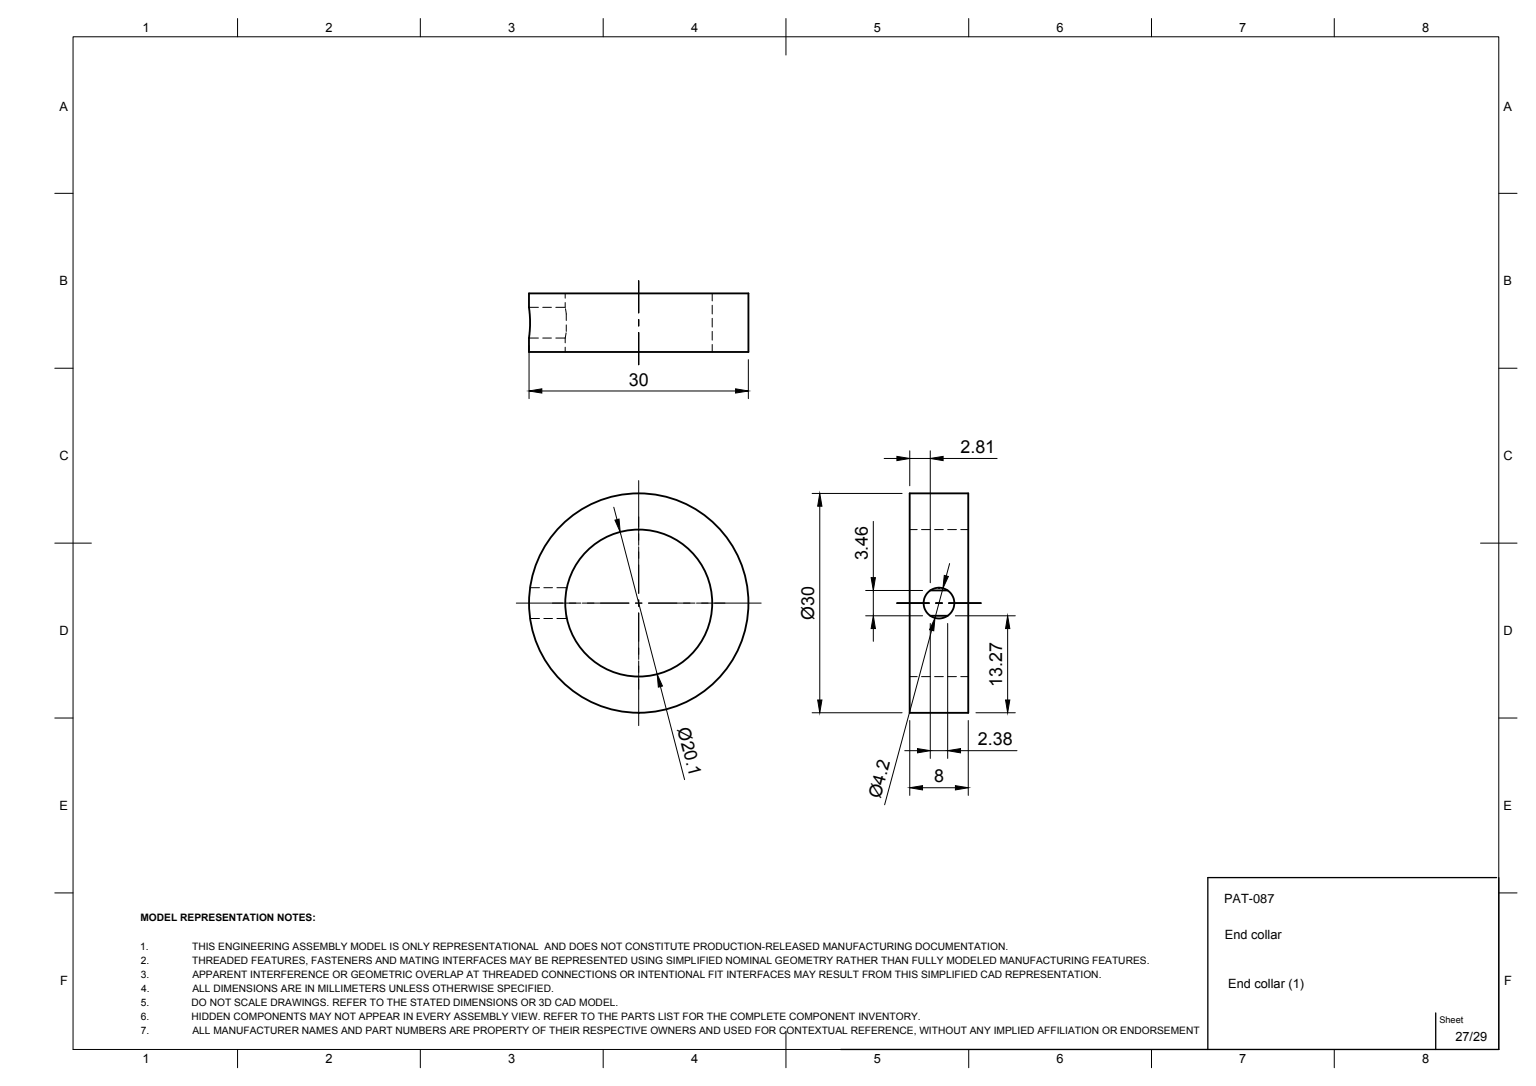
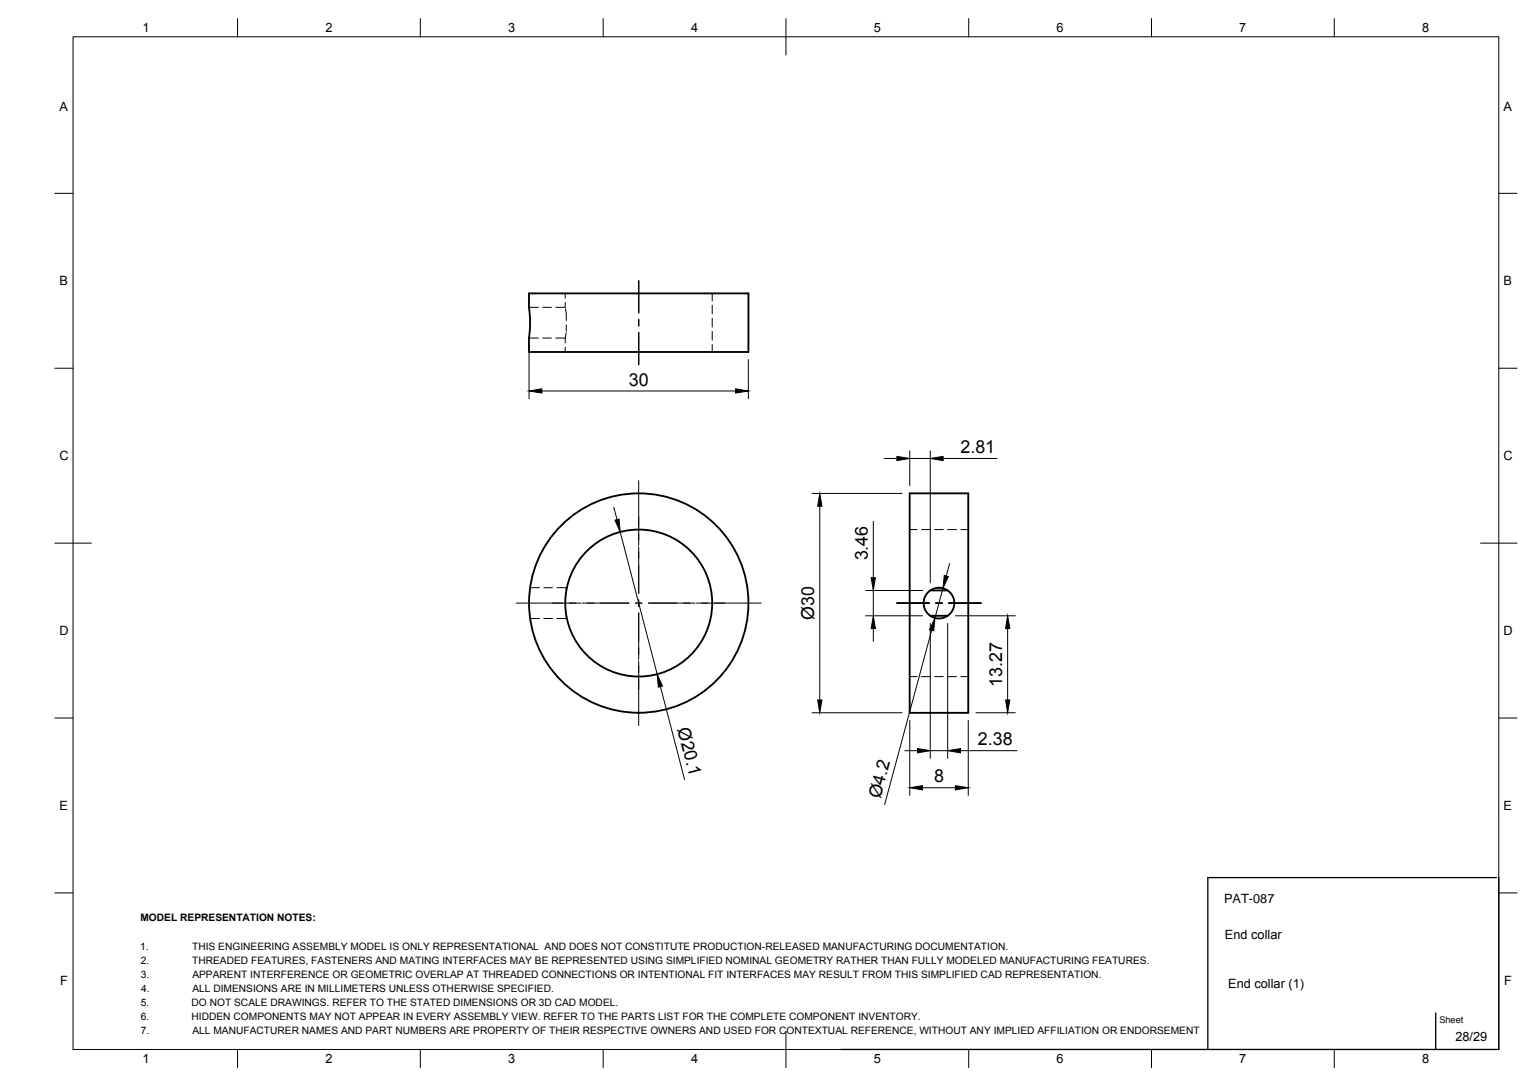
ISO-10303-21;
HEADER;
/* Generated by software containing ST-Developer
 * from STEP Tools, Inc. (www.steptools.com) 
 */

FILE_DESCRIPTION(
/* description */ ('Rigid flange shaft coupling assembly'),
/* implementation_level */ '2;1');

FILE_NAME(
/* name */ 'End collar.step',
/* time_stamp */ '2026-10-27T10:47:16-07:00',
/* author */ (''),
/* organization */ (''),
/* preprocessor_version */ 'ST-DEVELOPER v20.2',
/* originating_system */ 'Autodesk Translation Framework v15.17.0.0',
/* authorisation */ '');

FILE_SCHEMA (('AUTOMOTIVE_DESIGN { 1 0 10303 214 3 1 1 }'));
ENDSEC;

DATA;
#10=MECHANICAL_DESIGN_GEOMETRIC_PRESENTATION_REPRESENTATION('',(#419),#9141);
#332=B_SPLINE_CURVE_WITH_KNOTS('',3,(#8495,#8496,#8497,#8498,#8499,#8500,
#8501,#8502,#8503,#8504,#8505,#8506,#8507,#8508),.UNSPECIFIED.,.F.,.F.,
(4,2,2,2,2,2,4),(0.75600573798702,0.793568827564647,0.872922520054201,0.952276212543756,
1.03162990503331,1.11098359752287,1.14854668710049),.UNSPECIFIED.);
#333=B_SPLINE_CURVE_WITH_KNOTS('',3,(#8514,#8515,#8516,#8517,#8518,#8519,
#8520,#8521,#8522,#8523,#8524,#8525,#8526,#8527,#8528,#8529,#8530,#8531),
 .UNSPECIFIED.,.F.,.F.,(4,2,2,2,2,2,2,2,4),(0.,0.079216580773363,0.158433161546726,
0.23764869707457,0.316864232602414,0.396079768130259,0.475295303658103,
0.554511884431466,0.633728465204829),.UNSPECIFIED.);
#334=B_SPLINE_CURVE_WITH_KNOTS('',3,(#8532,#8533,#8534,#8535,#8536,#8537,
#8538,#8539,#8540,#8541,#8542,#8543,#8544,#8545,#8546,#8547,#8548,#8549),
 .UNSPECIFIED.,.F.,.F.,(4,2,2,2,2,2,2,2,4),(0.633728465204829,0.712945045978192,
0.792161626751555,0.871377162279399,0.950592697807243,1.02980823333509,
1.10902376886293,1.18824034963629,1.26745693040966),.UNSPECIFIED.);
#335=B_SPLINE_CURVE_WITH_KNOTS('',3,(#8552,#8553,#8554,#8555,#8556,#8557,
#8558,#8559,#8560,#8561,#8562,#8563,#8564,#8565),.UNSPECIFIED.,.F.,.F.,
(4,2,2,2,2,2,4),(0.121154929624515,0.158718019202143,0.238071711691697,
0.317425404181252,0.396779096670807,0.476132789160362,0.513695878737989),
 .UNSPECIFIED.);
#362=SHAPE_REPRESENTATION_RELATIONSHIP('SRR','None',#9298,#390);
#390=ADVANCED_BREP_SHAPE_REPRESENTATION('',(#447),#9133);
#419=STYLED_ITEM('',(#9486),#447);
#447=MANIFOLD_SOLID_BREP('Body1',#4774);
#555=FACE_BOUND('',#1309,.T.);
#556=FACE_BOUND('',#1311,.T.);
#557=FACE_BOUND('',#1313,.T.);
#558=FACE_BOUND('',#1315,.T.);
#685=PLANE('',#5446);
#686=PLANE('',#5451);
#687=PLANE('',#5458);
#688=PLANE('',#5459);
#931=FACE_OUTER_BOUND('',#1305,.T.);
#932=FACE_OUTER_BOUND('',#1306,.T.);
#933=FACE_OUTER_BOUND('',#1307,.T.);
#934=FACE_OUTER_BOUND('',#1308,.T.);
#935=FACE_OUTER_BOUND('',#1310,.T.);
#936=FACE_OUTER_BOUND('',#1312,.T.);
#937=FACE_OUTER_BOUND('',#1314,.T.);
#1305=EDGE_LOOP('',(#4047,#4048));
#1306=EDGE_LOOP('',(#4049,#4050,#4051,#4052,#4053,#4054,#4055,#4056,#4057));
#1307=EDGE_LOOP('',(#4058,#4059,#4060));
#1308=EDGE_LOOP('',(#4061,#4062,#4063,#4064));
#1309=EDGE_LOOP('',(#4065,#4066,#4067,#4068));
#1310=EDGE_LOOP('',(#4069,#4070,#4071,#4072));
#1311=EDGE_LOOP('',(#4073,#4074));
#1312=EDGE_LOOP('',(#4075));
#1313=EDGE_LOOP('',(#4076));
#1314=EDGE_LOOP('',(#4077));
#1315=EDGE_LOOP('',(#4078));
#1636=LINE('',#8491,#1981);
#1637=LINE('',#8512,#1982);
#1638=LINE('',#8567,#1983);
#1639=LINE('',#8572,#1984);
#1640=LINE('',#8578,#1985);
#1981=VECTOR('',#6581,1.);
#1982=VECTOR('',#6588,0.21);
#1983=VECTOR('',#6593,1.);
#1984=VECTOR('',#6598,1.005);
#1985=VECTOR('',#6605,1.5);
#2234=CIRCLE('',#5447,0.21);
#2235=CIRCLE('',#5449,0.21);
#2236=CIRCLE('',#5450,0.21);
#2237=CIRCLE('',#5453,1.005);
#2238=CIRCLE('',#5454,1.005);
#2239=CIRCLE('',#5456,1.5);
#2240=CIRCLE('',#5457,1.5);
#2551=VERTEX_POINT('',#8489);
#2552=VERTEX_POINT('',#8490);
#2553=VERTEX_POINT('',#8494);
#2554=VERTEX_POINT('',#8509);
#2555=VERTEX_POINT('',#8511);
#2556=VERTEX_POINT('',#8513);
#2557=VERTEX_POINT('',#8550);
#2558=VERTEX_POINT('',#8569);
#2559=VERTEX_POINT('',#8571);
#2560=VERTEX_POINT('',#8575);
#2561=VERTEX_POINT('',#8577);
#3067=EDGE_CURVE('',#2551,#2552,#1636,.T.);
#3068=EDGE_CURVE('',#2551,#2552,#2234,.T.);
#3069=EDGE_CURVE('',#2553,#2551,#332,.T.);
#3070=EDGE_CURVE('',#2554,#2553,#2235,.T.);
#3071=EDGE_CURVE('',#2554,#2555,#1637,.T.);
#3072=EDGE_CURVE('',#2556,#2555,#333,.T.);
#3073=EDGE_CURVE('',#2555,#2556,#334,.T.);
#3074=EDGE_CURVE('',#2557,#2554,#2236,.T.);
#3075=EDGE_CURVE('',#2552,#2557,#335,.T.);
#3076=EDGE_CURVE('',#2557,#2553,#1638,.T.);
#3077=EDGE_CURVE('',#2558,#2558,#2237,.T.);
#3078=EDGE_CURVE('',#2558,#2559,#1639,.T.);
#3079=EDGE_CURVE('',#2559,#2559,#2238,.T.);
#3080=EDGE_CURVE('',#2560,#2560,#2239,.T.);
#3081=EDGE_CURVE('',#2560,#2561,#1640,.T.);
#3082=EDGE_CURVE('',#2561,#2561,#2240,.T.);
#4047=ORIENTED_EDGE('',*,*,#3067,.F.);
#4048=ORIENTED_EDGE('',*,*,#3068,.T.);
#4049=ORIENTED_EDGE('',*,*,#3069,.F.);
#4050=ORIENTED_EDGE('',*,*,#3070,.F.);
#4051=ORIENTED_EDGE('',*,*,#3071,.T.);
#4052=ORIENTED_EDGE('',*,*,#3072,.F.);
#4053=ORIENTED_EDGE('',*,*,#3073,.F.);
#4054=ORIENTED_EDGE('',*,*,#3071,.F.);
#4055=ORIENTED_EDGE('',*,*,#3074,.F.);
#4056=ORIENTED_EDGE('',*,*,#3075,.F.);
#4057=ORIENTED_EDGE('',*,*,#3068,.F.);
#4058=ORIENTED_EDGE('',*,*,#3076,.F.);
#4059=ORIENTED_EDGE('',*,*,#3074,.T.);
#4060=ORIENTED_EDGE('',*,*,#3070,.T.);
#4061=ORIENTED_EDGE('',*,*,#3077,.F.);
#4062=ORIENTED_EDGE('',*,*,#3078,.T.);
#4063=ORIENTED_EDGE('',*,*,#3079,.T.);
#4064=ORIENTED_EDGE('',*,*,#3078,.F.);
#4065=ORIENTED_EDGE('',*,*,#3075,.T.);
#4066=ORIENTED_EDGE('',*,*,#3076,.T.);
#4067=ORIENTED_EDGE('',*,*,#3069,.T.);
#4068=ORIENTED_EDGE('',*,*,#3067,.T.);
#4069=ORIENTED_EDGE('',*,*,#3080,.F.);
#4070=ORIENTED_EDGE('',*,*,#3081,.T.);
#4071=ORIENTED_EDGE('',*,*,#3082,.T.);
#4072=ORIENTED_EDGE('',*,*,#3081,.F.);
#4073=ORIENTED_EDGE('',*,*,#3072,.T.);
#4074=ORIENTED_EDGE('',*,*,#3073,.T.);
#4075=ORIENTED_EDGE('',*,*,#3080,.T.);
#4076=ORIENTED_EDGE('',*,*,#3077,.T.);
#4077=ORIENTED_EDGE('',*,*,#3082,.F.);
#4078=ORIENTED_EDGE('',*,*,#3079,.F.);
#4466=CYLINDRICAL_SURFACE('',#5448,0.21);
#4467=CYLINDRICAL_SURFACE('',#5452,1.005);
#4468=CYLINDRICAL_SURFACE('',#5455,1.5);
#4667=ADVANCED_FACE('',(#931),#685,.T.);
#4668=ADVANCED_FACE('',(#932),#4466,.F.);
#4669=ADVANCED_FACE('',(#933),#686,.T.);
#4670=ADVANCED_FACE('',(#934,#555),#4467,.F.);
#4671=ADVANCED_FACE('',(#935,#556),#4468,.T.);
#4672=ADVANCED_FACE('',(#936,#557),#687,.T.);
#4673=ADVANCED_FACE('',(#937,#558),#688,.F.);
#4774=CLOSED_SHELL('',(#4667,#4668,#4669,#4670,#4671,#4672,#4673));
#5445=AXIS2_PLACEMENT_3D('',#8487,#6577,#6578);
#5446=AXIS2_PLACEMENT_3D('',#8488,#6579,#6580);
#5447=AXIS2_PLACEMENT_3D('',#8492,#6582,#6583);
#5448=AXIS2_PLACEMENT_3D('',#8493,#6584,#6585);
#5449=AXIS2_PLACEMENT_3D('',#8510,#6586,#6587);
#5450=AXIS2_PLACEMENT_3D('',#8551,#6589,#6590);
#5451=AXIS2_PLACEMENT_3D('',#8566,#6591,#6592);
#5452=AXIS2_PLACEMENT_3D('',#8568,#6594,#6595);
#5453=AXIS2_PLACEMENT_3D('',#8570,#6596,#6597);
#5454=AXIS2_PLACEMENT_3D('',#8573,#6599,#6600);
#5455=AXIS2_PLACEMENT_3D('',#8574,#6601,#6602);
#5456=AXIS2_PLACEMENT_3D('',#8576,#6603,#6604);
#5457=AXIS2_PLACEMENT_3D('',#8579,#6606,#6607);
#5458=AXIS2_PLACEMENT_3D('',#8580,#6608,#6609);
#5459=AXIS2_PLACEMENT_3D('',#8581,#6610,#6611);
#6577=DIRECTION('axis',(0.,0.,1.));
#6578=DIRECTION('refdir',(1.,0.,0.));
#6579=DIRECTION('center_axis',(0.,0.,1.));
#6580=DIRECTION('ref_axis',(1.,0.,0.));
#6581=DIRECTION('',(0.,1.,0.));
#6582=DIRECTION('center_axis',(0.,0.,1.));
#6583=DIRECTION('ref_axis',(1.,0.,0.));
#6584=DIRECTION('center_axis',(0.,0.,1.));
#6585=DIRECTION('ref_axis',(1.,0.,0.));
#6586=DIRECTION('center_axis',(0.,0.,1.));
#6587=DIRECTION('ref_axis',(1.,0.,0.));
#6588=DIRECTION('',(0.,0.,1.));
#6589=DIRECTION('center_axis',(0.,0.,1.));
#6590=DIRECTION('ref_axis',(1.,0.,0.));
#6591=DIRECTION('center_axis',(0.,0.,1.));
#6592=DIRECTION('ref_axis',(1.,0.,0.));
#6593=DIRECTION('',(0.,-1.,0.));
#6594=DIRECTION('center_axis',(0.,1.,0.));
#6595=DIRECTION('ref_axis',(1.,0.,0.));
#6596=DIRECTION('center_axis',(0.,-1.,0.));
#6597=DIRECTION('ref_axis',(1.,0.,0.));
#6598=DIRECTION('',(0.,-1.,0.));
#6599=DIRECTION('center_axis',(0.,-1.,0.));
#6600=DIRECTION('ref_axis',(1.,0.,0.));
#6601=DIRECTION('center_axis',(0.,1.,0.));
#6602=DIRECTION('ref_axis',(1.,0.,0.));
#6603=DIRECTION('center_axis',(0.,1.,0.));
#6604=DIRECTION('ref_axis',(1.,0.,0.));
#6605=DIRECTION('',(0.,-1.,0.));
#6606=DIRECTION('center_axis',(0.,1.,0.));
#6607=DIRECTION('ref_axis',(1.,0.,0.));
#6608=DIRECTION('center_axis',(0.,1.,0.));
#6609=DIRECTION('ref_axis',(1.,0.,0.));
#6610=DIRECTION('center_axis',(0.,1.,0.));
#6611=DIRECTION('ref_axis',(1.,0.,0.));
#8487=CARTESIAN_POINT('',(0.,0.,0.));
#8488=CARTESIAN_POINT('Origin',(0.,-1.25,7.52));
#8489=CARTESIAN_POINT('',(0.172988438920056,-1.36905880899792,7.52));
#8490=CARTESIAN_POINT('',(0.172988438920056,-1.13094119100209,7.52));
#8491=CARTESIAN_POINT('',(0.172988438920056,-1.65,7.52));
#8492=CARTESIAN_POINT('Origin',(0.,-1.25,7.52));
#8493=CARTESIAN_POINT('Origin',(0.,-1.25,7.52));
#8494=CARTESIAN_POINT('',(-0.172988438920056,-1.36905880899792,7.52));
#8495=CARTESIAN_POINT('Ctrl Pts',(-0.172988438920056,-1.36905880899792,
7.52));
#8496=CARTESIAN_POINT('Ctrl Pts',(-0.165594865311314,-1.37980142239529,
7.52129192197638));
#8497=CARTESIAN_POINT('Ctrl Pts',(-0.157297138725606,-1.38968770937274,
7.52265394943905));
#8498=CARTESIAN_POINT('Ctrl Pts',(-0.129892073845076,-1.41709277425327,
7.5267480843909));
#8499=CARTESIAN_POINT('Ctrl Pts',(-0.106330167759284,-1.43324205633295,
7.52969589327638));
#8500=CARTESIAN_POINT('Ctrl Pts',(-0.0546129046324105,-1.45469779396491,
7.53385029472357));
#8501=CARTESIAN_POINT('Ctrl Pts',(-0.0264512308298517,-1.46,7.535));
#8502=CARTESIAN_POINT('Ctrl Pts',(0.0264512308298516,-1.46,7.535));
#8503=CARTESIAN_POINT('Ctrl Pts',(0.0546129046324104,-1.45469779396491,
7.53385029472357));
#8504=CARTESIAN_POINT('Ctrl Pts',(0.106330167759284,-1.43324205633295,7.52969589327638));
#8505=CARTESIAN_POINT('Ctrl Pts',(0.129892073845076,-1.41709277425327,7.5267480843909));
#8506=CARTESIAN_POINT('Ctrl Pts',(0.157297138725606,-1.38968770937274,7.52265394943905));
#8507=CARTESIAN_POINT('Ctrl Pts',(0.165594865311315,-1.37980142239529,7.52129192197638));
#8508=CARTESIAN_POINT('Ctrl Pts',(0.172988438920056,-1.36905880899792,7.52));
#8509=CARTESIAN_POINT('',(-0.21,-1.25,7.52));
#8510=CARTESIAN_POINT('Origin',(0.,-1.25,7.52));
#8511=CARTESIAN_POINT('',(-0.21,-1.25,8.01522725533839));
#8512=CARTESIAN_POINT('',(-0.21,-1.25,7.52));
#8513=CARTESIAN_POINT('',(0.21,-1.25,8.01522725533839));
#8514=CARTESIAN_POINT('Ctrl Pts',(0.21,-1.25,8.01522725533839));
#8515=CARTESIAN_POINT('Ctrl Pts',(0.21,-1.27640552692445,8.01522725533839));
#8516=CARTESIAN_POINT('Ctrl Pts',(0.204715737269596,-1.30454707409071,8.01600415954412));
#8517=CARTESIAN_POINT('Ctrl Pts',(0.183273763036332,-1.35627626890513,8.01880073282317));
#8518=CARTESIAN_POINT('Ctrl Pts',(0.167117923970394,-1.37986692412796,8.02077897157582));
#8519=CARTESIAN_POINT('Ctrl Pts',(0.129867169887369,-1.41711767821098,8.02448481141327));
#8520=CARTESIAN_POINT('Ctrl Pts',(0.106276408305765,-1.43327371000135,8.02645455657129));
#8521=CARTESIAN_POINT('Ctrl Pts',(0.0545468514059001,-1.45471582482622,
8.02923165515645));
#8522=CARTESIAN_POINT('Ctrl Pts',(0.0264051785092814,-1.46,8.03));
#8523=CARTESIAN_POINT('Ctrl Pts',(-0.0264051785092814,-1.46,8.03));
#8524=CARTESIAN_POINT('Ctrl Pts',(-0.0545468514059,-1.45471582482622,8.02923165515645));
#8525=CARTESIAN_POINT('Ctrl Pts',(-0.106276408305765,-1.43327371000135,
8.02645455657129));
#8526=CARTESIAN_POINT('Ctrl Pts',(-0.129867169887369,-1.41711767821098,
8.02448481141327));
#8527=CARTESIAN_POINT('Ctrl Pts',(-0.167117923970394,-1.37986692412796,
8.02077897157582));
#8528=CARTESIAN_POINT('Ctrl Pts',(-0.183273763036331,-1.35627626890513,
8.01880073282317));
#8529=CARTESIAN_POINT('Ctrl Pts',(-0.204715737269596,-1.30454707409071,
8.01600415954412));
#8530=CARTESIAN_POINT('Ctrl Pts',(-0.21,-1.27640552692445,8.01522725533839));
#8531=CARTESIAN_POINT('Ctrl Pts',(-0.21,-1.25,8.01522725533839));
#8532=CARTESIAN_POINT('Ctrl Pts',(-0.21,-1.25,8.01522725533839));
#8533=CARTESIAN_POINT('Ctrl Pts',(-0.21,-1.22359447307555,8.01522725533839));
#8534=CARTESIAN_POINT('Ctrl Pts',(-0.204715737269596,-1.19545292590929,
8.01600415954412));
#8535=CARTESIAN_POINT('Ctrl Pts',(-0.183273763036332,-1.14372373109487,
8.01880073282317));
#8536=CARTESIAN_POINT('Ctrl Pts',(-0.167117923970394,-1.12013307587204,
8.02077897157582));
#8537=CARTESIAN_POINT('Ctrl Pts',(-0.129867169887369,-1.08288232178902,
8.02448481141327));
#8538=CARTESIAN_POINT('Ctrl Pts',(-0.106276408305765,-1.06672628999865,
8.02645455657129));
#8539=CARTESIAN_POINT('Ctrl Pts',(-0.0545468514059001,-1.04528417517378,
8.02923165515645));
#8540=CARTESIAN_POINT('Ctrl Pts',(-0.0264051785092814,-1.04,8.03));
#8541=CARTESIAN_POINT('Ctrl Pts',(0.0264051785092814,-1.04,8.03));
#8542=CARTESIAN_POINT('Ctrl Pts',(0.0545468514059002,-1.04528417517378,
8.02923165515645));
#8543=CARTESIAN_POINT('Ctrl Pts',(0.106276408305765,-1.06672628999865,8.02645455657129));
#8544=CARTESIAN_POINT('Ctrl Pts',(0.129867169887369,-1.08288232178902,8.02448481141327));
#8545=CARTESIAN_POINT('Ctrl Pts',(0.167117923970394,-1.12013307587204,8.02077897157582));
#8546=CARTESIAN_POINT('Ctrl Pts',(0.183273763036331,-1.14372373109487,8.01880073282317));
#8547=CARTESIAN_POINT('Ctrl Pts',(0.204715737269596,-1.19545292590929,8.01600415954412));
#8548=CARTESIAN_POINT('Ctrl Pts',(0.21,-1.22359447307555,8.01522725533839));
#8549=CARTESIAN_POINT('Ctrl Pts',(0.21,-1.25,8.01522725533839));
#8550=CARTESIAN_POINT('',(-0.172988438920056,-1.13094119100209,7.52));
#8551=CARTESIAN_POINT('Origin',(0.,-1.25,7.52));
#8552=CARTESIAN_POINT('Ctrl Pts',(0.172988438920056,-1.13094119100209,7.52));
#8553=CARTESIAN_POINT('Ctrl Pts',(0.165594865311315,-1.12019857760471,7.52129192197638));
#8554=CARTESIAN_POINT('Ctrl Pts',(0.157297138725606,-1.11031229062726,7.52265394943905));
#8555=CARTESIAN_POINT('Ctrl Pts',(0.129892073845076,-1.08290722574673,7.5267480843909));
#8556=CARTESIAN_POINT('Ctrl Pts',(0.106330167759284,-1.06675794366705,7.52969589327638));
#8557=CARTESIAN_POINT('Ctrl Pts',(0.0546129046324104,-1.04530220603509,
7.53385029472357));
#8558=CARTESIAN_POINT('Ctrl Pts',(0.0264512308298516,-1.04,7.535));
#8559=CARTESIAN_POINT('Ctrl Pts',(-0.0264512308298516,-1.04,7.535));
#8560=CARTESIAN_POINT('Ctrl Pts',(-0.0546129046324104,-1.04530220603509,
7.53385029472357));
#8561=CARTESIAN_POINT('Ctrl Pts',(-0.106330167759284,-1.06675794366705,
7.52969589327638));
#8562=CARTESIAN_POINT('Ctrl Pts',(-0.129892073845076,-1.08290722574673,
7.5267480843909));
#8563=CARTESIAN_POINT('Ctrl Pts',(-0.157297138725606,-1.11031229062726,
7.52265394943905));
#8564=CARTESIAN_POINT('Ctrl Pts',(-0.165594865311315,-1.12019857760471,
7.52129192197638));
#8565=CARTESIAN_POINT('Ctrl Pts',(-0.172988438920056,-1.13094119100209,
7.52));
#8566=CARTESIAN_POINT('Origin',(0.,-1.25,7.52));
#8567=CARTESIAN_POINT('',(-0.172988438920056,-1.65,7.52));
#8568=CARTESIAN_POINT('Origin',(0.,-1.65,6.53));
#8569=CARTESIAN_POINT('',(-1.005,-0.85,6.53));
#8570=CARTESIAN_POINT('Origin',(0.,-0.85,6.53));
#8571=CARTESIAN_POINT('',(-1.005,-1.65,6.53));
#8572=CARTESIAN_POINT('',(-1.005,-1.65,6.53));
#8573=CARTESIAN_POINT('Origin',(0.,-1.65,6.53));
#8574=CARTESIAN_POINT('Origin',(0.,-1.65,6.53));
#8575=CARTESIAN_POINT('',(-1.5,-0.85,6.53));
#8576=CARTESIAN_POINT('Origin',(0.,-0.85,6.53));
#8577=CARTESIAN_POINT('',(-1.5,-1.65,6.53));
#8578=CARTESIAN_POINT('',(-1.5,-1.65,6.53));
#8579=CARTESIAN_POINT('Origin',(0.,-1.65,6.53));
#8580=CARTESIAN_POINT('Origin',(0.,-0.85,6.53));
#8581=CARTESIAN_POINT('Origin',(0.,-1.65,6.53));
#9100=UNCERTAINTY_MEASURE_WITH_UNIT(LENGTH_MEASURE(0.001),#9142,
'DISTANCE_ACCURACY_VALUE',
'Maximum model space distance between geometric entities at asserted c
onnectivities');
#9108=UNCERTAINTY_MEASURE_WITH_UNIT(LENGTH_MEASURE(0.001),#9142,
'DISTANCE_ACCURACY_VALUE',
'Maximum model space distance between geometric entities at asserted c
onnectivities');
#9133=(
GEOMETRIC_REPRESENTATION_CONTEXT(3)
GLOBAL_UNCERTAINTY_ASSIGNED_CONTEXT((#9100))
GLOBAL_UNIT_ASSIGNED_CONTEXT((#9142,#9144,#9145))
REPRESENTATION_CONTEXT('','3D')
);
#9141=(
GEOMETRIC_REPRESENTATION_CONTEXT(3)
GLOBAL_UNCERTAINTY_ASSIGNED_CONTEXT((#9108))
GLOBAL_UNIT_ASSIGNED_CONTEXT((#9142,#9144,#9145))
REPRESENTATION_CONTEXT('','3D')
);
#9142=(
LENGTH_UNIT()
NAMED_UNIT(*)
SI_UNIT(.CENTI.,.METRE.)
);
#9144=(
NAMED_UNIT(*)
PLANE_ANGLE_UNIT()
SI_UNIT($,.RADIAN.)
);
#9145=(
NAMED_UNIT(*)
SI_UNIT($,.STERADIAN.)
SOLID_ANGLE_UNIT()
);
#9170=SHAPE_DEFINITION_REPRESENTATION(#9204,#9298);
#9204=PRODUCT_DEFINITION_SHAPE('',$,#9331);
#9298=SHAPE_REPRESENTATION('',(#5445),#9133);
#9306=PRODUCT_DEFINITION_CONTEXT('part definition',#9404,'design');
#9331=PRODUCT_DEFINITION('End collar','End collar',#9363,#9306);
#9363=PRODUCT_DEFINITION_FORMATION('',$,#9430);
#9404=APPLICATION_CONTEXT(
'Core Data for Automotive Mechanical Design Process');
#9405=PRODUCT_CONTEXT('part definition',#9404,'mechanical');
#9430=PRODUCT('End collar','End collar','End collar',(#9405));
#9480=COLOUR_RGB('Light Blue',0.38,0.62,0.78);
#9481=FILL_AREA_STYLE_COLOUR('',#9480);
#9482=FILL_AREA_STYLE('',(#9481));
#9483=SURFACE_STYLE_FILL_AREA(#9482);
#9484=SURFACE_SIDE_STYLE('',(#9483));
#9485=SURFACE_STYLE_USAGE(.BOTH.,#9484);
#9486=PRESENTATION_STYLE_ASSIGNMENT((#9485));
ENDSEC;
END-ISO-10303-21;
